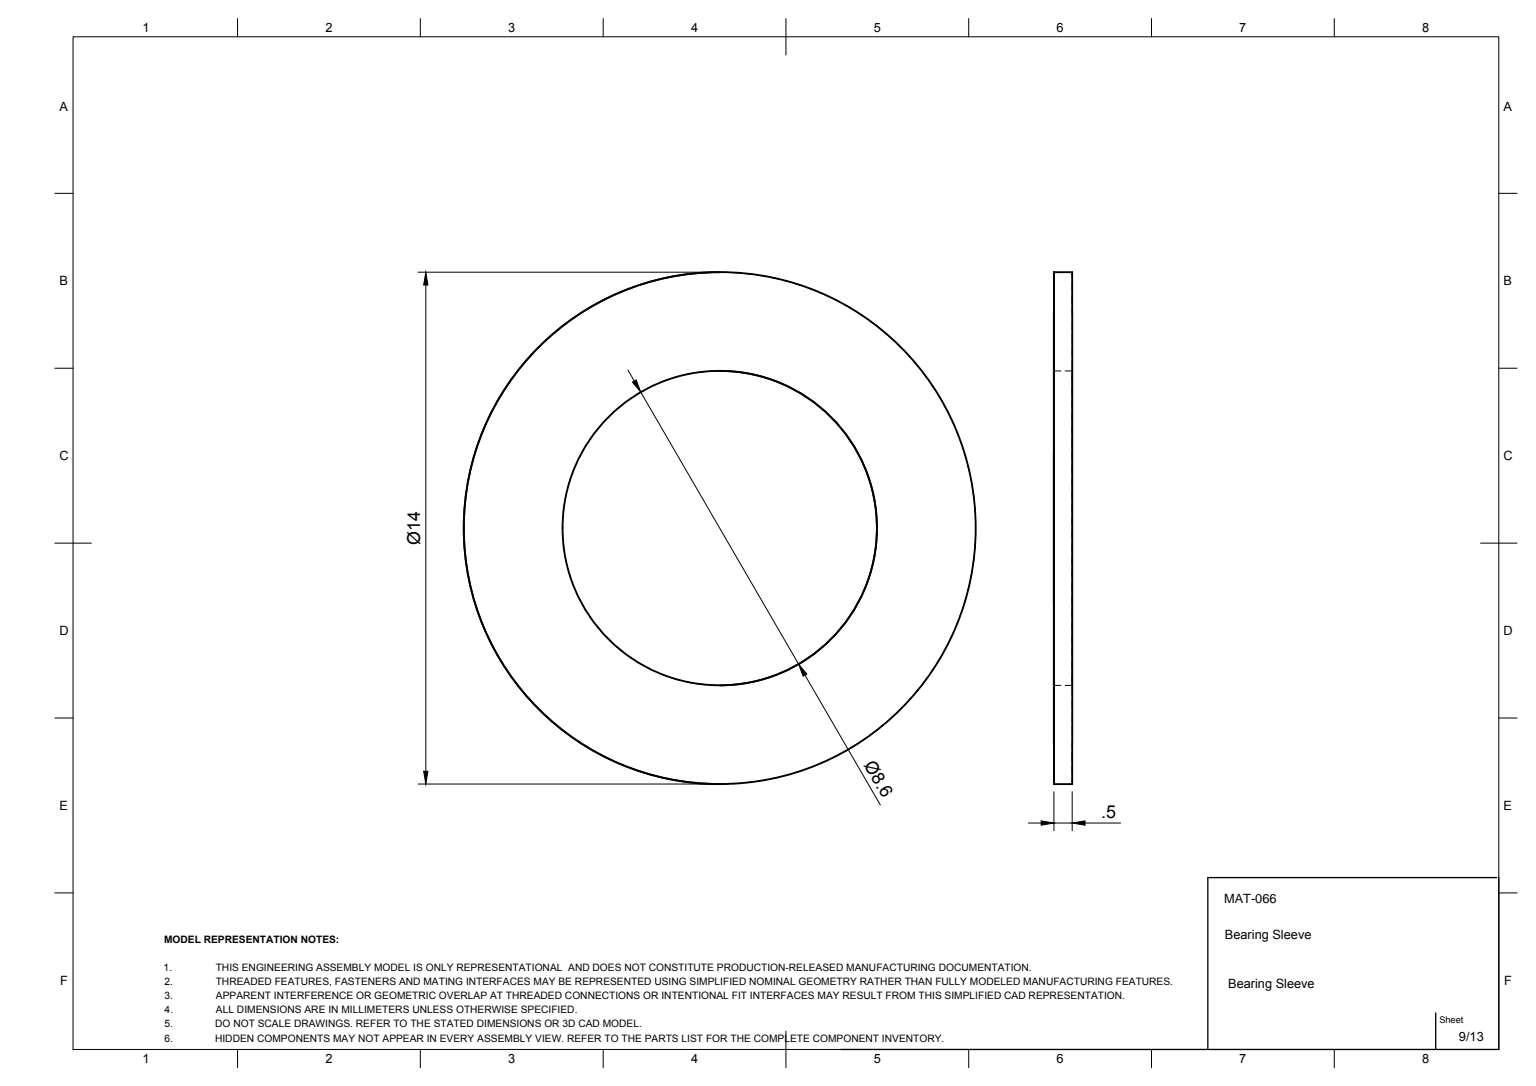
ISO-10303-21;
HEADER;
/* Generated by software containing ST-Developer
 * from STEP Tools, Inc. (www.steptools.com) 
 */

FILE_DESCRIPTION(
/* description */ ('CAx-IF Rec.Pracs.---Representation and Presentation of Product Manufa
cturing Information (PMI)---4.0---2014-10-13'),
/* implementation_level */ '2;1');

FILE_NAME(
/* name */ 'Bearing Sleeve.step',
/* time_stamp */ '2026-10-24T15:58:00-07:00',
/* author */ (''),
/* organization */ (''),
/* preprocessor_version */ 'ST-DEVELOPER v20.2',
/* originating_system */ 'Autodesk Translation Framework v15.17.0.0',
/* authorisation */ '');

FILE_SCHEMA (('AP242_MANAGED_MODEL_BASED_3D_ENGINEERING_MIM_LF { 1 0 10303 442 2 1 4 }'));
ENDSEC;

DATA;
#10=MECHANICAL_DESIGN_GEOMETRIC_PRESENTATION_REPRESENTATION('',(#133),#8944);
#115=SHAPE_REPRESENTATION_RELATIONSHIP('SRR','None',#8998,#124);
#124=ADVANCED_BREP_SHAPE_REPRESENTATION('',(#142),#8939);
#133=STYLED_ITEM('',(#9052),#142);
#142=MANIFOLD_SOLID_BREP('Body1',#5154);
#218=CYLINDRICAL_SURFACE('',#5690,0.007);
#219=CYLINDRICAL_SURFACE('',#5694,0.0043);
#288=FACE_BOUND('',#847,.T.);
#289=FACE_BOUND('',#850,.T.);
#527=FACE_OUTER_BOUND('',#846,.T.);
#528=FACE_OUTER_BOUND('',#848,.T.);
#529=FACE_OUTER_BOUND('',#849,.T.);
#530=FACE_OUTER_BOUND('',#851,.T.);
#846=EDGE_LOOP('',(#4541));
#847=EDGE_LOOP('',(#4542));
#848=EDGE_LOOP('',(#4543,#4544,#4545,#4546));
#849=EDGE_LOOP('',(#4547));
#850=EDGE_LOOP('',(#4548));
#851=EDGE_LOOP('',(#4549,#4550,#4551,#4552));
#1118=CIRCLE('',#5688,0.00700000000001);
#1119=CIRCLE('',#5689,0.00430000000001);
#1120=CIRCLE('',#5691,0.00700000000001);
#1121=CIRCLE('',#5693,0.00430000000001);
#1597=LINE('',#8715,#2052);
#1598=LINE('',#8720,#2053);
#2052=VECTOR('',#7108,0.007);
#2053=VECTOR('',#7115,0.0043);
#2504=VERTEX_POINT('',#8708);
#2505=VERTEX_POINT('',#8710);
#2506=VERTEX_POINT('',#8713);
#2507=VERTEX_POINT('',#8717);
#3191=EDGE_CURVE('',#2504,#2504,#1118,.T.);
#3192=EDGE_CURVE('',#2505,#2505,#1119,.T.);
#3193=EDGE_CURVE('',#2506,#2506,#1120,.T.);
#3194=EDGE_CURVE('',#2506,#2504,#1597,.T.);
#3195=EDGE_CURVE('',#2507,#2507,#1121,.T.);
#3196=EDGE_CURVE('',#2505,#2507,#1598,.T.);
#4541=ORIENTED_EDGE('',*,*,#3191,.F.);
#4542=ORIENTED_EDGE('',*,*,#3192,.T.);
#4543=ORIENTED_EDGE('',*,*,#3193,.F.);
#4544=ORIENTED_EDGE('',*,*,#3194,.T.);
#4545=ORIENTED_EDGE('',*,*,#3191,.T.);
#4546=ORIENTED_EDGE('',*,*,#3194,.F.);
#4547=ORIENTED_EDGE('',*,*,#3193,.T.);
#4548=ORIENTED_EDGE('',*,*,#3195,.F.);
#4549=ORIENTED_EDGE('',*,*,#3192,.F.);
#4550=ORIENTED_EDGE('',*,*,#3196,.T.);
#4551=ORIENTED_EDGE('',*,*,#3195,.T.);
#4552=ORIENTED_EDGE('',*,*,#3196,.F.);
#4861=PLANE('',#5687);
#4862=PLANE('',#5692);
#5100=ADVANCED_FACE('',(#527,#288),#4861,.T.);
#5101=ADVANCED_FACE('',(#528),#218,.T.);
#5102=ADVANCED_FACE('',(#529,#289),#4862,.T.);
#5103=ADVANCED_FACE('',(#530),#219,.F.);
#5154=CLOSED_SHELL('',(#5100,#5101,#5102,#5103));
#5686=AXIS2_PLACEMENT_3D('',#8706,#7096,#7097);
#5687=AXIS2_PLACEMENT_3D('',#8707,#7098,#7099);
#5688=AXIS2_PLACEMENT_3D('',#8709,#7100,#7101);
#5689=AXIS2_PLACEMENT_3D('',#8711,#7102,#7103);
#5690=AXIS2_PLACEMENT_3D('',#8712,#7104,#7105);
#5691=AXIS2_PLACEMENT_3D('',#8714,#7106,#7107);
#5692=AXIS2_PLACEMENT_3D('',#8716,#7109,#7110);
#5693=AXIS2_PLACEMENT_3D('',#8718,#7111,#7112);
#5694=AXIS2_PLACEMENT_3D('',#8719,#7113,#7114);
#7096=DIRECTION('axis',(0.,0.,1.));
#7097=DIRECTION('refdir',(1.,0.,0.));
#7098=DIRECTION('center_axis',(0.,-1.,0.));
#7099=DIRECTION('ref_axis',(0.,0.,-1.));
#7100=DIRECTION('center_axis',(0.,1.,0.));
#7101=DIRECTION('ref_axis',(1.,0.,0.));
#7102=DIRECTION('center_axis',(0.,1.,0.));
#7103=DIRECTION('ref_axis',(1.,0.,0.));
#7104=DIRECTION('center_axis',(0.,1.,0.));
#7105=DIRECTION('ref_axis',(0.,0.,1.));
#7106=DIRECTION('center_axis',(0.,1.,0.));
#7107=DIRECTION('ref_axis',(1.,0.,0.));
#7108=DIRECTION('',(0.,-1.,0.));
#7109=DIRECTION('center_axis',(0.,1.,0.));
#7110=DIRECTION('ref_axis',(1.,0.,0.));
#7111=DIRECTION('center_axis',(0.,1.,0.));
#7112=DIRECTION('ref_axis',(1.,0.,0.));
#7113=DIRECTION('center_axis',(0.,1.,0.));
#7114=DIRECTION('ref_axis',(0.,0.,1.));
#7115=DIRECTION('',(0.,1.,0.));
#8706=CARTESIAN_POINT('',(0.,0.,0.));
#8707=CARTESIAN_POINT('Origin',(0.,-0.0109999997541308,0.00699999995096662));
#8708=CARTESIAN_POINT('',(-8.57252759403147E-19,-0.0109999997541408,-0.00700000004903339));
#8709=CARTESIAN_POINT('Origin',(0.,-0.0109999997541408,-4.90433850849834E-11));
#8710=CARTESIAN_POINT('',(-5.26598123633362E-19,-0.0109999997541408,-0.00430000004903338));
#8711=CARTESIAN_POINT('Origin',(0.,-0.0109999997541408,-4.90433850849834E-11));
#8712=CARTESIAN_POINT('Origin',(0.,-0.0107499997597188,-4.90333850849834E-11));
#8713=CARTESIAN_POINT('',(-8.57252759403147E-19,-0.0104999997653167,-0.00700000004903339));
#8714=CARTESIAN_POINT('Origin',(0.,-0.0104999997653167,-4.90433850849834E-11));
#8715=CARTESIAN_POINT('',(-8.57252759403147E-19,-0.0107499997597188,-0.00700000004903339));
#8716=CARTESIAN_POINT('Origin',(0.,-0.0104999997653067,0.00429999995096661));
#8717=CARTESIAN_POINT('',(-5.26598123633362E-19,-0.0104999997653167,-0.00430000004903338));
#8718=CARTESIAN_POINT('Origin',(0.,-0.0104999997653167,-4.90433850849834E-11));
#8719=CARTESIAN_POINT('Origin',(0.,-0.0107499997597188,-4.90333850849834E-11));
#8720=CARTESIAN_POINT('',(-5.26598123633362E-19,-0.0107499997597188,-0.00430000004903338));
#8927=UNCERTAINTY_MEASURE_WITH_UNIT(LENGTH_MEASURE(1.E-5),#8945,
'DISTANCE_ACCURACY_VALUE',
'Maximum model space distance between geometric entities at asserted c
onnectivities');
#8932=UNCERTAINTY_MEASURE_WITH_UNIT(LENGTH_MEASURE(1.E-5),#8945,
'DISTANCE_ACCURACY_VALUE',
'Maximum model space distance between geometric entities at asserted c
onnectivities');
#8939=(
GEOMETRIC_REPRESENTATION_CONTEXT(3)
GLOBAL_UNCERTAINTY_ASSIGNED_CONTEXT((#8927))
GLOBAL_UNIT_ASSIGNED_CONTEXT((#8945,#8946,#8947))
REPRESENTATION_CONTEXT('','3D')
);
#8944=(
GEOMETRIC_REPRESENTATION_CONTEXT(3)
GLOBAL_UNCERTAINTY_ASSIGNED_CONTEXT((#8932))
GLOBAL_UNIT_ASSIGNED_CONTEXT((#8945,#8946,#8947))
REPRESENTATION_CONTEXT('','3D')
);
#8945=(
LENGTH_UNIT()
NAMED_UNIT(*)
SI_UNIT($,.METRE.)
);
#8946=(
NAMED_UNIT(*)
PLANE_ANGLE_UNIT()
SI_UNIT($,.RADIAN.)
);
#8947=(
NAMED_UNIT(*)
SI_UNIT($,.STERADIAN.)
SOLID_ANGLE_UNIT()
);
#8954=SHAPE_DEFINITION_REPRESENTATION(#8965,#8998);
#8965=PRODUCT_DEFINITION_SHAPE('',$,#9010);
#8998=SHAPE_REPRESENTATION('',(#5686),#8939);
#9003=PRODUCT_DEFINITION_CONTEXT('part definition',#9038,'design');
#9010=PRODUCT_DEFINITION('Bearing Sleeve','Bearing Sleeve',#9021,#9003);
#9021=PRODUCT_DEFINITION_FORMATION('',$,#9046);
#9038=APPLICATION_CONTEXT('Managed model based 3d engineering');
#9039=PRODUCT_CONTEXT('part definition',#9038,'mechanical');
#9046=PRODUCT('Bearing Sleeve','Bearing Sleeve',
'LEGAL AND USAGE DISCLAIMER: this Data/Model is provided \X2\201C\X0\A
S IS\X2\201D\X0\ for informational and representational only. It is a 
geometric approximation and is NOT engineered, certified, or guarantee
d for dimensional accuracy, exact tolerances, or production-level prec
ision. Vendor disclaims all implied warranties including fitness for a
 particular purpose. DO NOT USE FOR DIRECT PHYSICAL MANUFACTURING, AUT
OMATED PRODUCTION, OR SAFETY-CRITICAL SYSTEMS without independent engi
neering verification and resolution of any design discrepancies.',(#9039));
#9052=PRESENTATION_STYLE_ASSIGNMENT((#9057));
#9057=SURFACE_STYLE_USAGE(.BOTH.,#9062);
#9062=SURFACE_SIDE_STYLE('',(#9067));
#9067=SURFACE_STYLE_FILL_AREA(#9072);
#9072=FILL_AREA_STYLE('Opaque(25,25,25)',(#9077));
#9077=FILL_AREA_STYLE_COLOUR('Opaque(25,25,25)',#9082);
#9082=COLOUR_RGB('Opaque(25,25,25)',0.0980392156862745,0.0980392156862745,
0.0980392156862745);
ENDSEC;
END-ISO-10303-21;
